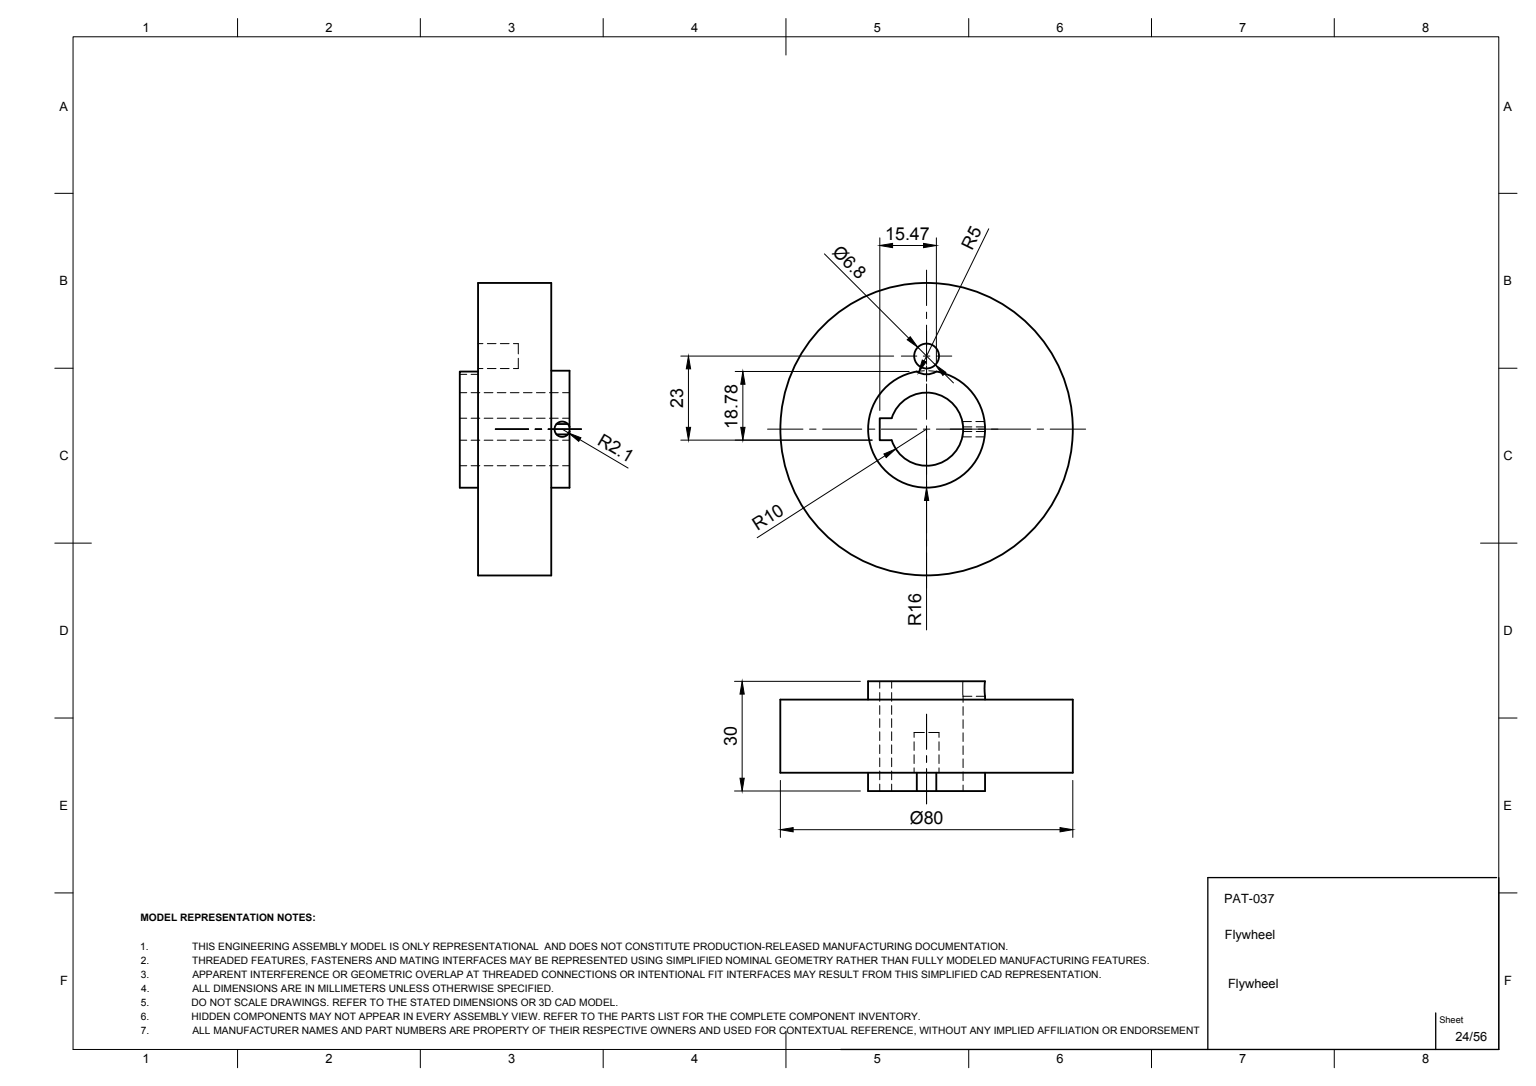
ISO-10303-21;
HEADER;
/* Generated by software containing ST-Developer
 * from STEP Tools, Inc. (www.steptools.com) 
 */

FILE_DESCRIPTION(
/* description */ ('Flywheel Crank-Slider'),
/* implementation_level */ '2;1');

FILE_NAME(
/* name */ 'Flywheel.step',
/* time_stamp */ '2026-10-28T03:23:13-07:00',
/* author */ (''),
/* organization */ (''),
/* preprocessor_version */ 'ST-DEVELOPER v20.2',
/* originating_system */ 'Autodesk Translation Framework v15.17.0.0',
/* authorisation */ '');

FILE_SCHEMA (('AUTOMOTIVE_DESIGN { 1 0 10303 214 3 1 1 }'));
ENDSEC;

DATA;
#10=MECHANICAL_DESIGN_GEOMETRIC_PRESENTATION_REPRESENTATION('',(#694),#17322);
#489=B_SPLINE_CURVE_WITH_KNOTS('',3,(#15673,#15674,#15675,#15676,#15677,
#15678,#15679,#15680,#15681,#15682),.UNSPECIFIED.,.F.,.F.,(4,2,2,2,4),(0.168950313426779,
0.238079516586307,0.317435737633656,0.396791958681006,0.465921161840534),
 .UNSPECIFIED.);
#490=B_SPLINE_CURVE_WITH_KNOTS('',3,(#15686,#15687,#15688,#15689,#15690,
#15691),.UNSPECIFIED.,.F.,.F.,(4,2,4),(1.01510699658258,1.03166343394832,
1.10079263710785),.UNSPECIFIED.);
#491=B_SPLINE_CURVE_WITH_KNOTS('',3,(#15695,#15696,#15697,#15698,#15699,
#15700,#15701,#15702,#15703,#15704,#15705,#15706,#15707,#15708,#15709,#15710,
#15711,#15712,#15713,#15714,#15715,#15716,#15717,#15718,#15719,#15720,#15721,
#15722,#15723,#15724,#15725,#15726,#15727,#15728,#15729),.UNSPECIFIED.,
 .F.,.F.,(4,2,2,2,2,2,2,2,2,2,2,2,3,2,2,2,4),(0.379554434981269,0.396011596624156,
0.475213593758045,0.554416396369289,0.633619198980533,0.712822001591777,
0.792024804203021,0.87122680133691,0.950428798470799,1.02963079560469,1.10883279273858,
1.18803559534982,1.26723839796107,1.34644120057231,1.42564400318355,1.50484600031744,
1.52130316196033),.UNSPECIFIED.);
#492=B_SPLINE_CURVE_WITH_KNOTS('',3,(#15732,#15733,#15734,#15735,#15736,
#15737),.UNSPECIFIED.,.F.,.F.,(4,2,4),(0.803821788694091,0.872950991853619,
0.889507429219361),.UNSPECIFIED.);
#589=SHAPE_REPRESENTATION_RELATIONSHIP('SRR','None',#17587,#641);
#641=ADVANCED_BREP_SHAPE_REPRESENTATION('',(#751),#17291);
#694=STYLED_ITEM('',(#17945),#751);
#751=MANIFOLD_SOLID_BREP('Body1',#9076);
#918=FACE_BOUND('',#2290,.T.);
#919=FACE_BOUND('',#2301,.T.);
#920=FACE_BOUND('',#2302,.T.);
#921=FACE_BOUND('',#2304,.T.);
#1191=PLANE('',#10240);
#1192=PLANE('',#10246);
#1193=PLANE('',#10247);
#1194=PLANE('',#10251);
#1195=PLANE('',#10255);
#1196=PLANE('',#10256);
#1197=PLANE('',#10257);
#1198=PLANE('',#10258);
#1199=PLANE('',#10261);
#1200=PLANE('',#10269);
#1620=FACE_OUTER_BOUND('',#2288,.T.);
#1621=FACE_OUTER_BOUND('',#2289,.T.);
#1622=FACE_OUTER_BOUND('',#2291,.T.);
#1623=FACE_OUTER_BOUND('',#2292,.T.);
#1624=FACE_OUTER_BOUND('',#2293,.T.);
#1625=FACE_OUTER_BOUND('',#2294,.T.);
#1626=FACE_OUTER_BOUND('',#2295,.T.);
#1627=FACE_OUTER_BOUND('',#2296,.T.);
#1628=FACE_OUTER_BOUND('',#2297,.T.);
#1629=FACE_OUTER_BOUND('',#2298,.T.);
#1630=FACE_OUTER_BOUND('',#2299,.T.);
#1631=FACE_OUTER_BOUND('',#2300,.T.);
#1632=FACE_OUTER_BOUND('',#2303,.T.);
#1633=FACE_OUTER_BOUND('',#2305,.T.);
#1634=FACE_OUTER_BOUND('',#2306,.T.);
#1635=FACE_OUTER_BOUND('',#2307,.T.);
#1636=FACE_OUTER_BOUND('',#2308,.T.);
#2288=EDGE_LOOP('',(#7384,#7385,#7386,#7387));
#2289=EDGE_LOOP('',(#7388,#7389));
#2290=EDGE_LOOP('',(#7390,#7391,#7392,#7393));
#2291=EDGE_LOOP('',(#7394,#7395,#7396,#7397));
#2292=EDGE_LOOP('',(#7398));
#2293=EDGE_LOOP('',(#7399,#7400));
#2294=EDGE_LOOP('',(#7401,#7402,#7403,#7404,#7405,#7406,#7407,#7408));
#2295=EDGE_LOOP('',(#7409,#7410));
#2296=EDGE_LOOP('',(#7411,#7412,#7413,#7414,#7415,#7416,#7417,#7418,#7419,
#7420));
#2297=EDGE_LOOP('',(#7421,#7422,#7423,#7424));
#2298=EDGE_LOOP('',(#7425,#7426,#7427,#7428));
#2299=EDGE_LOOP('',(#7429,#7430,#7431,#7432));
#2300=EDGE_LOOP('',(#7433));
#2301=EDGE_LOOP('',(#7434));
#2302=EDGE_LOOP('',(#7435,#7436));
#2303=EDGE_LOOP('',(#7437));
#2304=EDGE_LOOP('',(#7438));
#2305=EDGE_LOOP('',(#7439,#7440,#7441,#7442));
#2306=EDGE_LOOP('',(#7443,#7444,#7445,#7446,#7447,#7448));
#2307=EDGE_LOOP('',(#7449,#7450,#7451,#7452));
#2308=EDGE_LOOP('',(#7453,#7454,#7455,#7456,#7457,#7458,#7459,#7460,#7461));
#2995=LINE('',#15643,#3606);
#2996=LINE('',#15647,#3607);
#2997=LINE('',#15653,#3608);
#2998=LINE('',#15655,#3609);
#2999=LINE('',#15657,#3610);
#3000=LINE('',#15663,#3611);
#3001=LINE('',#15669,#3612);
#3002=LINE('',#15693,#3613);
#3003=LINE('',#15731,#3614);
#3004=LINE('',#15739,#3615);
#3005=LINE('',#15743,#3616);
#3006=LINE('',#15745,#3617);
#3007=LINE('',#15749,#3618);
#3008=LINE('',#15750,#3619);
#3009=LINE('',#15753,#3620);
#3010=LINE('',#15754,#3621);
#3011=LINE('',#15756,#3622);
#3012=LINE('',#15767,#3623);
#3013=LINE('',#15770,#3624);
#3606=VECTOR('',#12315,1.);
#3607=VECTOR('',#12318,1.);
#3608=VECTOR('',#12325,1.);
#3609=VECTOR('',#12326,1.);
#3610=VECTOR('',#12327,1.);
#3611=VECTOR('',#12334,0.34);
#3612=VECTOR('',#12341,1.);
#3613=VECTOR('',#12348,1.);
#3614=VECTOR('',#12349,1.);
#3615=VECTOR('',#12352,1.);
#3616=VECTOR('',#12357,1.);
#3617=VECTOR('',#12358,1.);
#3618=VECTOR('',#12363,1.);
#3619=VECTOR('',#12364,1.);
#3620=VECTOR('',#12367,1.);
#3621=VECTOR('',#12368,1.);
#3622=VECTOR('',#12371,1.);
#3623=VECTOR('',#12386,4.);
#3624=VECTOR('',#12389,1.6);
#4058=CIRCLE('',#10238,0.5);
#4059=CIRCLE('',#10239,0.5);
#4060=CIRCLE('',#10241,1.6);
#4061=CIRCLE('',#10242,1.);
#4062=CIRCLE('',#10244,0.34);
#4063=CIRCLE('',#10245,0.34);
#4064=CIRCLE('',#10248,0.21);
#4065=CIRCLE('',#10250,0.21);
#4066=CIRCLE('',#10253,1.);
#4067=CIRCLE('',#10254,1.);
#4068=CIRCLE('',#10259,4.);
#4069=CIRCLE('',#10260,1.6);
#4070=CIRCLE('',#10262,4.);
#4071=CIRCLE('',#10263,1.6);
#4072=CIRCLE('',#10266,1.6);
#4073=CIRCLE('',#10267,1.6);
#4695=VERTEX_POINT('',#15641);
#4696=VERTEX_POINT('',#15642);
#4697=VERTEX_POINT('',#15644);
#4698=VERTEX_POINT('',#15646);
#4699=VERTEX_POINT('',#15651);
#4700=VERTEX_POINT('',#15652);
#4701=VERTEX_POINT('',#15654);
#4702=VERTEX_POINT('',#15656);
#4703=VERTEX_POINT('',#15660);
#4704=VERTEX_POINT('',#15662);
#4705=VERTEX_POINT('',#15667);
#4706=VERTEX_POINT('',#15668);
#4707=VERTEX_POINT('',#15672);
#4708=VERTEX_POINT('',#15683);
#4709=VERTEX_POINT('',#15685);
#4710=VERTEX_POINT('',#15692);
#4711=VERTEX_POINT('',#15694);
#4712=VERTEX_POINT('',#15730);
#4713=VERTEX_POINT('',#15741);
#4714=VERTEX_POINT('',#15744);
#4715=VERTEX_POINT('',#15748);
#4716=VERTEX_POINT('',#15752);
#4717=VERTEX_POINT('',#15758);
#4718=VERTEX_POINT('',#15762);
#4719=VERTEX_POINT('',#15764);
#4720=VERTEX_POINT('',#15769);
#5649=EDGE_CURVE('',#4695,#4696,#2995,.T.);
#5650=EDGE_CURVE('',#4697,#4695,#4058,.T.);
#5651=EDGE_CURVE('',#4698,#4697,#2996,.T.);
#5652=EDGE_CURVE('',#4696,#4698,#4059,.T.);
#5653=EDGE_CURVE('',#4698,#4696,#4060,.T.);
#5654=EDGE_CURVE('',#4699,#4700,#2997,.T.);
#5655=EDGE_CURVE('',#4700,#4701,#2998,.T.);
#5656=EDGE_CURVE('',#4701,#4702,#2999,.T.);
#5657=EDGE_CURVE('',#4702,#4699,#4061,.T.);
#5658=EDGE_CURVE('',#4703,#4703,#4062,.T.);
#5659=EDGE_CURVE('',#4703,#4704,#3000,.T.);
#5660=EDGE_CURVE('',#4704,#4704,#4063,.T.);
#5661=EDGE_CURVE('',#4705,#4706,#3001,.T.);
#5662=EDGE_CURVE('',#4705,#4706,#4064,.T.);
#5663=EDGE_CURVE('',#4707,#4705,#489,.T.);
#5664=EDGE_CURVE('',#4708,#4707,#4065,.T.);
#5665=EDGE_CURVE('',#4709,#4708,#490,.T.);
#5666=EDGE_CURVE('',#4710,#4709,#3002,.T.);
#5667=EDGE_CURVE('',#4711,#4710,#491,.T.);
#5668=EDGE_CURVE('',#4712,#4711,#3003,.T.);
#5669=EDGE_CURVE('',#4706,#4712,#492,.T.);
#5670=EDGE_CURVE('',#4708,#4707,#3004,.T.);
#5671=EDGE_CURVE('',#4712,#4713,#4066,.T.);
#5672=EDGE_CURVE('',#4713,#4699,#3005,.T.);
#5673=EDGE_CURVE('',#4702,#4714,#3006,.T.);
#5674=EDGE_CURVE('',#4714,#4709,#4067,.T.);
#5675=EDGE_CURVE('',#4715,#4713,#3007,.T.);
#5676=EDGE_CURVE('',#4715,#4700,#3008,.T.);
#5677=EDGE_CURVE('',#4716,#4715,#3009,.T.);
#5678=EDGE_CURVE('',#4716,#4701,#3010,.T.);
#5679=EDGE_CURVE('',#4714,#4716,#3011,.T.);
#5680=EDGE_CURVE('',#4717,#4717,#4068,.T.);
#5681=EDGE_CURVE('',#4697,#4695,#4069,.T.);
#5682=EDGE_CURVE('',#4718,#4718,#4070,.T.);
#5683=EDGE_CURVE('',#4719,#4719,#4071,.T.);
#5684=EDGE_CURVE('',#4717,#4718,#3012,.T.);
#5685=EDGE_CURVE('',#4719,#4720,#3013,.T.);
#5686=EDGE_CURVE('',#4720,#4711,#4072,.T.);
#5687=EDGE_CURVE('',#4710,#4720,#4073,.T.);
#7384=ORIENTED_EDGE('',*,*,#5649,.F.);
#7385=ORIENTED_EDGE('',*,*,#5650,.F.);
#7386=ORIENTED_EDGE('',*,*,#5651,.F.);
#7387=ORIENTED_EDGE('',*,*,#5652,.F.);
#7388=ORIENTED_EDGE('',*,*,#5652,.T.);
#7389=ORIENTED_EDGE('',*,*,#5653,.T.);
#7390=ORIENTED_EDGE('',*,*,#5654,.T.);
#7391=ORIENTED_EDGE('',*,*,#5655,.T.);
#7392=ORIENTED_EDGE('',*,*,#5656,.T.);
#7393=ORIENTED_EDGE('',*,*,#5657,.T.);
#7394=ORIENTED_EDGE('',*,*,#5658,.F.);
#7395=ORIENTED_EDGE('',*,*,#5659,.T.);
#7396=ORIENTED_EDGE('',*,*,#5660,.F.);
#7397=ORIENTED_EDGE('',*,*,#5659,.F.);
#7398=ORIENTED_EDGE('',*,*,#5658,.T.);
#7399=ORIENTED_EDGE('',*,*,#5661,.F.);
#7400=ORIENTED_EDGE('',*,*,#5662,.T.);
#7401=ORIENTED_EDGE('',*,*,#5663,.F.);
#7402=ORIENTED_EDGE('',*,*,#5664,.F.);
#7403=ORIENTED_EDGE('',*,*,#5665,.F.);
#7404=ORIENTED_EDGE('',*,*,#5666,.F.);
#7405=ORIENTED_EDGE('',*,*,#5667,.F.);
#7406=ORIENTED_EDGE('',*,*,#5668,.F.);
#7407=ORIENTED_EDGE('',*,*,#5669,.F.);
#7408=ORIENTED_EDGE('',*,*,#5662,.F.);
#7409=ORIENTED_EDGE('',*,*,#5670,.F.);
#7410=ORIENTED_EDGE('',*,*,#5664,.T.);
#7411=ORIENTED_EDGE('',*,*,#5665,.T.);
#7412=ORIENTED_EDGE('',*,*,#5670,.T.);
#7413=ORIENTED_EDGE('',*,*,#5663,.T.);
#7414=ORIENTED_EDGE('',*,*,#5661,.T.);
#7415=ORIENTED_EDGE('',*,*,#5669,.T.);
#7416=ORIENTED_EDGE('',*,*,#5671,.T.);
#7417=ORIENTED_EDGE('',*,*,#5672,.T.);
#7418=ORIENTED_EDGE('',*,*,#5657,.F.);
#7419=ORIENTED_EDGE('',*,*,#5673,.T.);
#7420=ORIENTED_EDGE('',*,*,#5674,.T.);
#7421=ORIENTED_EDGE('',*,*,#5675,.F.);
#7422=ORIENTED_EDGE('',*,*,#5676,.T.);
#7423=ORIENTED_EDGE('',*,*,#5654,.F.);
#7424=ORIENTED_EDGE('',*,*,#5672,.F.);
#7425=ORIENTED_EDGE('',*,*,#5677,.F.);
#7426=ORIENTED_EDGE('',*,*,#5678,.T.);
#7427=ORIENTED_EDGE('',*,*,#5655,.F.);
#7428=ORIENTED_EDGE('',*,*,#5676,.F.);
#7429=ORIENTED_EDGE('',*,*,#5679,.F.);
#7430=ORIENTED_EDGE('',*,*,#5673,.F.);
#7431=ORIENTED_EDGE('',*,*,#5656,.F.);
#7432=ORIENTED_EDGE('',*,*,#5678,.F.);
#7433=ORIENTED_EDGE('',*,*,#5680,.T.);
#7434=ORIENTED_EDGE('',*,*,#5660,.T.);
#7435=ORIENTED_EDGE('',*,*,#5681,.F.);
#7436=ORIENTED_EDGE('',*,*,#5650,.T.);
#7437=ORIENTED_EDGE('',*,*,#5682,.F.);
#7438=ORIENTED_EDGE('',*,*,#5683,.F.);
#7439=ORIENTED_EDGE('',*,*,#5680,.F.);
#7440=ORIENTED_EDGE('',*,*,#5684,.T.);
#7441=ORIENTED_EDGE('',*,*,#5682,.T.);
#7442=ORIENTED_EDGE('',*,*,#5684,.F.);
#7443=ORIENTED_EDGE('',*,*,#5683,.T.);
#7444=ORIENTED_EDGE('',*,*,#5685,.T.);
#7445=ORIENTED_EDGE('',*,*,#5686,.T.);
#7446=ORIENTED_EDGE('',*,*,#5667,.T.);
#7447=ORIENTED_EDGE('',*,*,#5687,.T.);
#7448=ORIENTED_EDGE('',*,*,#5685,.F.);
#7449=ORIENTED_EDGE('',*,*,#5649,.T.);
#7450=ORIENTED_EDGE('',*,*,#5653,.F.);
#7451=ORIENTED_EDGE('',*,*,#5651,.T.);
#7452=ORIENTED_EDGE('',*,*,#5681,.T.);
#7453=ORIENTED_EDGE('',*,*,#5666,.T.);
#7454=ORIENTED_EDGE('',*,*,#5674,.F.);
#7455=ORIENTED_EDGE('',*,*,#5679,.T.);
#7456=ORIENTED_EDGE('',*,*,#5677,.T.);
#7457=ORIENTED_EDGE('',*,*,#5675,.T.);
#7458=ORIENTED_EDGE('',*,*,#5671,.F.);
#7459=ORIENTED_EDGE('',*,*,#5668,.T.);
#7460=ORIENTED_EDGE('',*,*,#5686,.F.);
#7461=ORIENTED_EDGE('',*,*,#5687,.F.);
#8432=CYLINDRICAL_SURFACE('',#10237,0.5);
#8433=CYLINDRICAL_SURFACE('',#10243,0.34);
#8434=CYLINDRICAL_SURFACE('',#10249,0.21);
#8435=CYLINDRICAL_SURFACE('',#10252,1.);
#8436=CYLINDRICAL_SURFACE('',#10264,4.);
#8437=CYLINDRICAL_SURFACE('',#10265,1.6);
#8438=CYLINDRICAL_SURFACE('',#10268,1.6);
#8811=ADVANCED_FACE('',(#1620),#8432,.F.);
#8812=ADVANCED_FACE('',(#1621,#918),#1191,.T.);
#8813=ADVANCED_FACE('',(#1622),#8433,.F.);
#8814=ADVANCED_FACE('',(#1623),#1192,.T.);
#8815=ADVANCED_FACE('',(#1624),#1193,.T.);
#8816=ADVANCED_FACE('',(#1625),#8434,.F.);
#8817=ADVANCED_FACE('',(#1626),#1194,.T.);
#8818=ADVANCED_FACE('',(#1627),#8435,.F.);
#8819=ADVANCED_FACE('',(#1628),#1195,.F.);
#8820=ADVANCED_FACE('',(#1629),#1196,.F.);
#8821=ADVANCED_FACE('',(#1630),#1197,.F.);
#8822=ADVANCED_FACE('',(#1631,#919,#920),#1198,.T.);
#8823=ADVANCED_FACE('',(#1632,#921),#1199,.F.);
#8824=ADVANCED_FACE('',(#1633),#8436,.T.);
#8825=ADVANCED_FACE('',(#1634),#8437,.T.);
#8826=ADVANCED_FACE('',(#1635),#8438,.T.);
#8827=ADVANCED_FACE('',(#1636),#1200,.F.);
#9076=CLOSED_SHELL('',(#8811,#8812,#8813,#8814,#8815,#8816,#8817,#8818,
#8819,#8820,#8821,#8822,#8823,#8824,#8825,#8826,#8827));
#10236=AXIS2_PLACEMENT_3D('',#15639,#12311,#12312);
#10237=AXIS2_PLACEMENT_3D('',#15640,#12313,#12314);
#10238=AXIS2_PLACEMENT_3D('',#15645,#12316,#12317);
#10239=AXIS2_PLACEMENT_3D('',#15648,#12319,#12320);
#10240=AXIS2_PLACEMENT_3D('',#15649,#12321,#12322);
#10241=AXIS2_PLACEMENT_3D('',#15650,#12323,#12324);
#10242=AXIS2_PLACEMENT_3D('',#15658,#12328,#12329);
#10243=AXIS2_PLACEMENT_3D('',#15659,#12330,#12331);
#10244=AXIS2_PLACEMENT_3D('',#15661,#12332,#12333);
#10245=AXIS2_PLACEMENT_3D('',#15664,#12335,#12336);
#10246=AXIS2_PLACEMENT_3D('',#15665,#12337,#12338);
#10247=AXIS2_PLACEMENT_3D('',#15666,#12339,#12340);
#10248=AXIS2_PLACEMENT_3D('',#15670,#12342,#12343);
#10249=AXIS2_PLACEMENT_3D('',#15671,#12344,#12345);
#10250=AXIS2_PLACEMENT_3D('',#15684,#12346,#12347);
#10251=AXIS2_PLACEMENT_3D('',#15738,#12350,#12351);
#10252=AXIS2_PLACEMENT_3D('',#15740,#12353,#12354);
#10253=AXIS2_PLACEMENT_3D('',#15742,#12355,#12356);
#10254=AXIS2_PLACEMENT_3D('',#15746,#12359,#12360);
#10255=AXIS2_PLACEMENT_3D('',#15747,#12361,#12362);
#10256=AXIS2_PLACEMENT_3D('',#15751,#12365,#12366);
#10257=AXIS2_PLACEMENT_3D('',#15755,#12369,#12370);
#10258=AXIS2_PLACEMENT_3D('',#15757,#12372,#12373);
#10259=AXIS2_PLACEMENT_3D('',#15759,#12374,#12375);
#10260=AXIS2_PLACEMENT_3D('',#15760,#12376,#12377);
#10261=AXIS2_PLACEMENT_3D('',#15761,#12378,#12379);
#10262=AXIS2_PLACEMENT_3D('',#15763,#12380,#12381);
#10263=AXIS2_PLACEMENT_3D('',#15765,#12382,#12383);
#10264=AXIS2_PLACEMENT_3D('',#15766,#12384,#12385);
#10265=AXIS2_PLACEMENT_3D('',#15768,#12387,#12388);
#10266=AXIS2_PLACEMENT_3D('',#15771,#12390,#12391);
#10267=AXIS2_PLACEMENT_3D('',#15772,#12392,#12393);
#10268=AXIS2_PLACEMENT_3D('',#15773,#12394,#12395);
#10269=AXIS2_PLACEMENT_3D('',#15774,#12396,#12397);
#12311=DIRECTION('axis',(0.,0.,1.));
#12312=DIRECTION('refdir',(1.,0.,0.));
#12313=DIRECTION('center_axis',(0.,1.,0.));
#12314=DIRECTION('ref_axis',(-1.,0.,1.22464679914735E-16));
#12315=DIRECTION('',(0.,1.,0.));
#12316=DIRECTION('center_axis',(0.,1.,0.));
#12317=DIRECTION('ref_axis',(1.,0.,0.));
#12318=DIRECTION('',(0.,-1.,0.));
#12319=DIRECTION('center_axis',(0.,-1.,0.));
#12320=DIRECTION('ref_axis',(1.,0.,0.));
#12321=DIRECTION('center_axis',(0.,1.,0.));
#12322=DIRECTION('ref_axis',(1.,0.,0.));
#12323=DIRECTION('center_axis',(0.,1.,0.));
#12324=DIRECTION('ref_axis',(1.,0.,0.));
#12325=DIRECTION('',(0.,0.,-1.));
#12326=DIRECTION('',(1.,0.,0.));
#12327=DIRECTION('',(0.,0.,1.));
#12328=DIRECTION('center_axis',(0.,-1.,0.));
#12329=DIRECTION('ref_axis',(1.,0.,0.));
#12330=DIRECTION('center_axis',(0.,1.,0.));
#12331=DIRECTION('ref_axis',(1.,0.,0.));
#12332=DIRECTION('center_axis',(0.,1.,0.));
#12333=DIRECTION('ref_axis',(1.,0.,0.));
#12334=DIRECTION('',(0.,1.,0.));
#12335=DIRECTION('center_axis',(0.,-1.,0.));
#12336=DIRECTION('ref_axis',(1.,0.,0.));
#12337=DIRECTION('center_axis',(0.,1.,0.));
#12338=DIRECTION('ref_axis',(1.,0.,0.));
#12339=DIRECTION('center_axis',(0.,0.,1.));
#12340=DIRECTION('ref_axis',(1.,0.,0.));
#12341=DIRECTION('',(0.,-1.,0.));
#12342=DIRECTION('center_axis',(0.,0.,1.));
#12343=DIRECTION('ref_axis',(1.,0.,0.));
#12344=DIRECTION('center_axis',(0.,0.,1.));
#12345=DIRECTION('ref_axis',(5.0532154980743E-16,1.,0.));
#12346=DIRECTION('center_axis',(0.,0.,1.));
#12347=DIRECTION('ref_axis',(1.,0.,0.));
#12348=DIRECTION('',(0.,0.,-1.));
#12349=DIRECTION('',(0.,0.,1.));
#12350=DIRECTION('center_axis',(0.,0.,1.));
#12351=DIRECTION('ref_axis',(1.,0.,0.));
#12352=DIRECTION('',(0.,1.,0.));
#12353=DIRECTION('center_axis',(0.,1.,0.));
#12354=DIRECTION('ref_axis',(6.12323399573677E-17,0.,1.));
#12355=DIRECTION('center_axis',(0.,-1.,0.));
#12356=DIRECTION('ref_axis',(1.,0.,0.));
#12357=DIRECTION('',(0.,1.,0.));
#12358=DIRECTION('',(0.,-1.,0.));
#12359=DIRECTION('center_axis',(0.,-1.,0.));
#12360=DIRECTION('ref_axis',(1.,0.,0.));
#12361=DIRECTION('center_axis',(-1.,0.,0.));
#12362=DIRECTION('ref_axis',(0.,0.,1.));
#12363=DIRECTION('',(0.,0.,1.));
#12364=DIRECTION('',(0.,1.,0.));
#12365=DIRECTION('center_axis',(0.,0.,-1.));
#12366=DIRECTION('ref_axis',(-1.,0.,0.));
#12367=DIRECTION('',(-1.,0.,0.));
#12368=DIRECTION('',(0.,1.,0.));
#12369=DIRECTION('center_axis',(1.,0.,0.));
#12370=DIRECTION('ref_axis',(0.,0.,-1.));
#12371=DIRECTION('',(0.,0.,-1.));
#12372=DIRECTION('center_axis',(0.,1.,0.));
#12373=DIRECTION('ref_axis',(1.,0.,0.));
#12374=DIRECTION('center_axis',(0.,1.,0.));
#12375=DIRECTION('ref_axis',(1.,0.,0.));
#12376=DIRECTION('center_axis',(0.,1.,0.));
#12377=DIRECTION('ref_axis',(1.,0.,0.));
#12378=DIRECTION('center_axis',(0.,1.,0.));
#12379=DIRECTION('ref_axis',(1.,0.,0.));
#12380=DIRECTION('center_axis',(0.,1.,0.));
#12381=DIRECTION('ref_axis',(1.,0.,0.));
#12382=DIRECTION('center_axis',(0.,-1.,0.));
#12383=DIRECTION('ref_axis',(1.,0.,0.));
#12384=DIRECTION('center_axis',(0.,1.,0.));
#12385=DIRECTION('ref_axis',(1.,0.,0.));
#12386=DIRECTION('',(0.,-1.,0.));
#12387=DIRECTION('center_axis',(0.,1.,0.));
#12388=DIRECTION('ref_axis',(1.,0.,0.));
#12389=DIRECTION('',(0.,-1.,0.));
#12390=DIRECTION('center_axis',(0.,1.,0.));
#12391=DIRECTION('ref_axis',(1.,0.,0.));
#12392=DIRECTION('center_axis',(0.,1.,0.));
#12393=DIRECTION('ref_axis',(1.,0.,0.));
#12394=DIRECTION('center_axis',(0.,1.,0.));
#12395=DIRECTION('ref_axis',(-1.,0.,1.22464679914735E-16));
#12396=DIRECTION('center_axis',(0.,1.,0.));
#12397=DIRECTION('ref_axis',(1.,0.,0.));
#15639=CARTESIAN_POINT('',(0.,0.,0.));
#15640=CARTESIAN_POINT('Origin',(2.,1.,10.));
#15641=CARTESIAN_POINT('',(1.5775,1.,10.2673831520496));
#15642=CARTESIAN_POINT('',(1.5775,1.5,10.2673831520496));
#15643=CARTESIAN_POINT('',(1.5775,1.,10.2673831520496));
#15644=CARTESIAN_POINT('',(1.5775,1.,9.73261684795036));
#15645=CARTESIAN_POINT('Origin',(2.,1.,10.));
#15646=CARTESIAN_POINT('',(1.5775,1.5,9.73261684795036));
#15647=CARTESIAN_POINT('',(1.5775,1.,9.73261684795036));
#15648=CARTESIAN_POINT('Origin',(2.,1.5,10.));
#15649=CARTESIAN_POINT('Origin',(0.,1.5,10.));
#15650=CARTESIAN_POINT('Origin',(0.,1.5,10.));
#15651=CARTESIAN_POINT('',(-0.3,1.5,9.04606079858305));
#15652=CARTESIAN_POINT('',(-0.3,1.5,8.72));
#15653=CARTESIAN_POINT('',(-0.3,1.5,9.36));
#15654=CARTESIAN_POINT('',(0.3,1.5,8.72));
#15655=CARTESIAN_POINT('',(0.15,1.5,8.72));
#15656=CARTESIAN_POINT('',(0.3,1.5,9.04606079858305));
#15657=CARTESIAN_POINT('',(0.3,1.5,10.));
#15658=CARTESIAN_POINT('Origin',(0.,1.5,10.));
#15659=CARTESIAN_POINT('Origin',(2.,-0.1,10.));
#15660=CARTESIAN_POINT('',(1.66,-0.1,10.));
#15661=CARTESIAN_POINT('Origin',(2.,-0.1,10.));
#15662=CARTESIAN_POINT('',(1.66,1.,10.));
#15663=CARTESIAN_POINT('',(1.66,-0.1,10.));
#15664=CARTESIAN_POINT('Origin',(2.,1.,10.));
#15665=CARTESIAN_POINT('Origin',(2.,-0.1,10.));
#15666=CARTESIAN_POINT('Origin',(0.,-1.3,10.99));
#15667=CARTESIAN_POINT('',(-0.141067359796645,-1.14443650813895,10.99));
#15668=CARTESIAN_POINT('',(-0.141067359796645,-1.45556349186105,10.99));
#15669=CARTESIAN_POINT('',(-0.141067359796645,-1.5,10.99));
#15670=CARTESIAN_POINT('Origin',(0.,-1.3,10.99));
#15671=CARTESIAN_POINT('Origin',(0.,-1.3,10.99));
#15672=CARTESIAN_POINT('',(0.141067359796645,-1.14443650813895,10.99));
#15673=CARTESIAN_POINT('Ctrl Pts',(0.141067359796645,-1.14443650813895,
10.99));
#15674=CARTESIAN_POINT('Ctrl Pts',(0.123818356698215,-1.1287948476368,10.9924578498245));
#15675=CARTESIAN_POINT('Ctrl Pts',(0.102998643109694,-1.11537595666898,
10.9949381930495));
#15676=CARTESIAN_POINT('Ctrl Pts',(0.054614114398353,-1.09530253627557,
10.9988444923724));
#15677=CARTESIAN_POINT('Ctrl Pts',(0.0264520736824499,-1.09,11.));
#15678=CARTESIAN_POINT('Ctrl Pts',(-0.0264520736824498,-1.09,11.));
#15679=CARTESIAN_POINT('Ctrl Pts',(-0.0546141143983528,-1.09530253627557,
10.9988444923724));
#15680=CARTESIAN_POINT('Ctrl Pts',(-0.102998643109694,-1.11537595666898,
10.9949381930495));
#15681=CARTESIAN_POINT('Ctrl Pts',(-0.123818356698214,-1.1287948476368,
10.9924578498245));
#15682=CARTESIAN_POINT('Ctrl Pts',(-0.141067359796645,-1.14443650813895,
10.99));
#15683=CARTESIAN_POINT('',(0.141067359796645,-1.45556349186105,10.99));
#15684=CARTESIAN_POINT('Origin',(0.,-1.3,10.99));
#15685=CARTESIAN_POINT('',(0.0640312423743287,-1.5,10.9979478944314));
#15686=CARTESIAN_POINT('Ctrl Pts',(0.0640312423743287,-1.5,10.9979478944314));
#15687=CARTESIAN_POINT('Ctrl Pts',(0.0695863834759532,-1.49822148706849,
10.9975914604048));
#15688=CARTESIAN_POINT('Ctrl Pts',(0.0750776578932034,-1.49620769804413,
10.9971923790166));
#15689=CARTESIAN_POINT('Ctrl Pts',(0.102998643109694,-1.48462404333102,
10.9949381930495));
#15690=CARTESIAN_POINT('Ctrl Pts',(0.123818356698214,-1.4712051523632,10.9924578498245));
#15691=CARTESIAN_POINT('Ctrl Pts',(0.141067359796645,-1.45556349186105,
10.99));
#15692=CARTESIAN_POINT('',(0.0640312423743287,-1.5,11.5987182365883));
#15693=CARTESIAN_POINT('',(0.0640312423743287,-1.5,10.99));
#15694=CARTESIAN_POINT('',(-0.0640312423743287,-1.5,11.5987182365883));
#15695=CARTESIAN_POINT('Ctrl Pts',(-0.0640312423743287,-1.5,11.5987182365883));
#15696=CARTESIAN_POINT('Ctrl Pts',(-0.0695623721690265,-1.49822917443756,
11.5984967059243));
#15697=CARTESIAN_POINT('Ctrl Pts',(-0.0750312749053373,-1.49622475645458,
11.5982488123351));
#15698=CARTESIAN_POINT('Ctrl Pts',(-0.106271159541076,-1.48327680083123,
11.5966769093301));
#15699=CARTESIAN_POINT('Ctrl Pts',(-0.129864750292352,-1.467120097806,11.5948307595328));
#15700=CARTESIAN_POINT('Ctrl Pts',(-0.167120287247804,-1.42986456085055,
11.5913581688701));
#15701=CARTESIAN_POINT('Ctrl Pts',(-0.183276841782292,-1.4062710523005,
11.5895050296478));
#15702=CARTESIAN_POINT('Ctrl Pts',(-0.20471752266132,-1.35454055536511,
11.586886062954));
#15703=CARTESIAN_POINT('Ctrl Pts',(-0.21,-1.32640093420375,11.5861588823318));
#15704=CARTESIAN_POINT('Ctrl Pts',(-0.21,-1.27359906579625,11.5861588823318));
#15705=CARTESIAN_POINT('Ctrl Pts',(-0.20471752266132,-1.24545944463489,
11.586886062954));
#15706=CARTESIAN_POINT('Ctrl Pts',(-0.183276841782292,-1.1937289476995,
11.5895050296478));
#15707=CARTESIAN_POINT('Ctrl Pts',(-0.167120287247804,-1.17013543914945,
11.5913581688701));
#15708=CARTESIAN_POINT('Ctrl Pts',(-0.129864750292352,-1.132879902194,11.5948307595328));
#15709=CARTESIAN_POINT('Ctrl Pts',(-0.106271159541076,-1.11672319916877,
11.5966769093301));
#15710=CARTESIAN_POINT('Ctrl Pts',(-0.0545403836274686,-1.0952824096556,
11.5992798562698));
#15711=CARTESIAN_POINT('Ctrl Pts',(-0.0264006657112965,-1.09,11.6));
#15712=CARTESIAN_POINT('Ctrl Pts',(0.0264006657112964,-1.09,11.6));
#15713=CARTESIAN_POINT('Ctrl Pts',(0.0545403836274687,-1.0952824096556,
11.5992798562698));
#15714=CARTESIAN_POINT('Ctrl Pts',(0.106271159541076,-1.11672319916877,
11.5966769093301));
#15715=CARTESIAN_POINT('Ctrl Pts',(0.129864750292352,-1.132879902194,11.5948307595328));
#15716=CARTESIAN_POINT('Ctrl Pts',(0.167120287247804,-1.17013543914945,
11.5913581688701));
#15717=CARTESIAN_POINT('Ctrl Pts',(0.183276841782292,-1.1937289476995,11.5895050296478));
#15718=CARTESIAN_POINT('Ctrl Pts',(0.20471752266132,-1.24545944463489,11.586886062954));
#15719=CARTESIAN_POINT('Ctrl Pts',(0.21,-1.27359906579625,11.5861588823318));
#15720=CARTESIAN_POINT('Ctrl Pts',(0.21,-1.3,11.5861588823318));
#15721=CARTESIAN_POINT('Ctrl Pts',(0.21,-1.32640093420375,11.5861588823318));
#15722=CARTESIAN_POINT('Ctrl Pts',(0.20471752266132,-1.35454055536511,11.586886062954));
#15723=CARTESIAN_POINT('Ctrl Pts',(0.183276841782292,-1.4062710523005,11.5895050296478));
#15724=CARTESIAN_POINT('Ctrl Pts',(0.167120287247804,-1.42986456085055,
11.5913581688701));
#15725=CARTESIAN_POINT('Ctrl Pts',(0.129864750292352,-1.467120097806,11.5948307595328));
#15726=CARTESIAN_POINT('Ctrl Pts',(0.106271159541076,-1.48327680083123,
11.5966769093301));
#15727=CARTESIAN_POINT('Ctrl Pts',(0.0750312749053373,-1.49622475645458,
11.5982488123351));
#15728=CARTESIAN_POINT('Ctrl Pts',(0.0695623721690265,-1.49822917443756,
11.5984967059243));
#15729=CARTESIAN_POINT('Ctrl Pts',(0.0640312423743287,-1.5,11.5987182365883));
#15730=CARTESIAN_POINT('',(-0.0640312423743287,-1.5,10.9979478944314));
#15731=CARTESIAN_POINT('',(-0.0640312423743287,-1.5,10.99));
#15732=CARTESIAN_POINT('Ctrl Pts',(-0.141067359796645,-1.45556349186105,
10.99));
#15733=CARTESIAN_POINT('Ctrl Pts',(-0.123818356698214,-1.4712051523632,
10.9924578498245));
#15734=CARTESIAN_POINT('Ctrl Pts',(-0.102998643109694,-1.48462404333102,
10.9949381930495));
#15735=CARTESIAN_POINT('Ctrl Pts',(-0.0750776578932034,-1.49620769804413,
10.9971923790166));
#15736=CARTESIAN_POINT('Ctrl Pts',(-0.0695863834759533,-1.49822148706849,
10.9975914604048));
#15737=CARTESIAN_POINT('Ctrl Pts',(-0.0640312423743287,-1.5,10.9979478944314));
#15738=CARTESIAN_POINT('Origin',(0.,-1.3,10.99));
#15739=CARTESIAN_POINT('',(0.141067359796645,-1.5,10.99));
#15740=CARTESIAN_POINT('Origin',(0.,-1.5,10.));
#15741=CARTESIAN_POINT('',(-0.3,-1.5,9.04606079858305));
#15742=CARTESIAN_POINT('Origin',(0.,-1.5,10.));
#15743=CARTESIAN_POINT('',(-0.3,-1.5,9.04606079858305));
#15744=CARTESIAN_POINT('',(0.3,-1.5,9.04606079858305));
#15745=CARTESIAN_POINT('',(0.3,-1.5,9.04606079858305));
#15746=CARTESIAN_POINT('Origin',(0.,-1.5,10.));
#15747=CARTESIAN_POINT('Origin',(-0.3,-1.6,8.72));
#15748=CARTESIAN_POINT('',(-0.3,-1.5,8.72));
#15749=CARTESIAN_POINT('',(-0.3,-1.5,9.36));
#15750=CARTESIAN_POINT('',(-0.3,-1.6,8.72));
#15751=CARTESIAN_POINT('Origin',(0.3,-1.6,8.72));
#15752=CARTESIAN_POINT('',(0.3,-1.5,8.72));
#15753=CARTESIAN_POINT('',(0.15,-1.5,8.72));
#15754=CARTESIAN_POINT('',(0.3,-1.6,8.72));
#15755=CARTESIAN_POINT('Origin',(0.3,-1.6,10.));
#15756=CARTESIAN_POINT('',(0.3,-1.5,10.));
#15757=CARTESIAN_POINT('Origin',(0.,1.,10.));
#15758=CARTESIAN_POINT('',(-4.,1.,10.));
#15759=CARTESIAN_POINT('Origin',(0.,1.,10.));
#15760=CARTESIAN_POINT('Origin',(0.,1.,10.));
#15761=CARTESIAN_POINT('Origin',(0.,-1.,10.));
#15762=CARTESIAN_POINT('',(-4.,-1.,10.));
#15763=CARTESIAN_POINT('Origin',(0.,-1.,10.));
#15764=CARTESIAN_POINT('',(-1.6,-1.,10.));
#15765=CARTESIAN_POINT('Origin',(0.,-1.,10.));
#15766=CARTESIAN_POINT('Origin',(0.,-1.,10.));
#15767=CARTESIAN_POINT('',(-4.,-1.,10.));
#15768=CARTESIAN_POINT('Origin',(0.,-1.5,10.));
#15769=CARTESIAN_POINT('',(-1.6,-1.5,10.));
#15770=CARTESIAN_POINT('',(-1.6,-1.5,10.));
#15771=CARTESIAN_POINT('Origin',(0.,-1.5,10.));
#15772=CARTESIAN_POINT('Origin',(0.,-1.5,10.));
#15773=CARTESIAN_POINT('Origin',(0.,-1.5,10.));
#15774=CARTESIAN_POINT('Origin',(0.,-1.5,10.));
#17230=UNCERTAINTY_MEASURE_WITH_UNIT(LENGTH_MEASURE(0.001),#17323,
'DISTANCE_ACCURACY_VALUE',
'Maximum model space distance between geometric entities at asserted c
onnectivities');
#17261=UNCERTAINTY_MEASURE_WITH_UNIT(LENGTH_MEASURE(0.001),#17323,
'DISTANCE_ACCURACY_VALUE',
'Maximum model space distance between geometric entities at asserted c
onnectivities');
#17291=(
GEOMETRIC_REPRESENTATION_CONTEXT(3)
GLOBAL_UNCERTAINTY_ASSIGNED_CONTEXT((#17230))
GLOBAL_UNIT_ASSIGNED_CONTEXT((#17323,#17325,#17326))
REPRESENTATION_CONTEXT('','3D')
);
#17322=(
GEOMETRIC_REPRESENTATION_CONTEXT(3)
GLOBAL_UNCERTAINTY_ASSIGNED_CONTEXT((#17261))
GLOBAL_UNIT_ASSIGNED_CONTEXT((#17323,#17325,#17326))
REPRESENTATION_CONTEXT('','3D')
);
#17323=(
LENGTH_UNIT()
NAMED_UNIT(*)
SI_UNIT(.CENTI.,.METRE.)
);
#17325=(
NAMED_UNIT(*)
PLANE_ANGLE_UNIT()
SI_UNIT($,.RADIAN.)
);
#17326=(
NAMED_UNIT(*)
SI_UNIT($,.STERADIAN.)
SOLID_ANGLE_UNIT()
);
#17356=SHAPE_DEFINITION_REPRESENTATION(#17418,#17587);
#17418=PRODUCT_DEFINITION_SHAPE('',$,#17648);
#17587=SHAPE_REPRESENTATION('',(#10236),#17291);
#17618=PRODUCT_DEFINITION_CONTEXT('part definition',#17800,'design');
#17648=PRODUCT_DEFINITION('Flywheel','Flywheel',#17708,#17618);
#17708=PRODUCT_DEFINITION_FORMATION('',$,#17831);
#17800=APPLICATION_CONTEXT(
'Core Data for Automotive Mechanical Design Process');
#17801=PRODUCT_CONTEXT('part definition',#17800,'mechanical');
#17831=PRODUCT('Flywheel','Flywheel','Flywheel',(#17801));
#17939=COLOUR_RGB('Off White',0.89,0.88,0.83);
#17940=FILL_AREA_STYLE_COLOUR('',#17939);
#17941=FILL_AREA_STYLE('',(#17940));
#17942=SURFACE_STYLE_FILL_AREA(#17941);
#17943=SURFACE_SIDE_STYLE('',(#17942));
#17944=SURFACE_STYLE_USAGE(.BOTH.,#17943);
#17945=PRESENTATION_STYLE_ASSIGNMENT((#17944));
ENDSEC;
END-ISO-10303-21;
